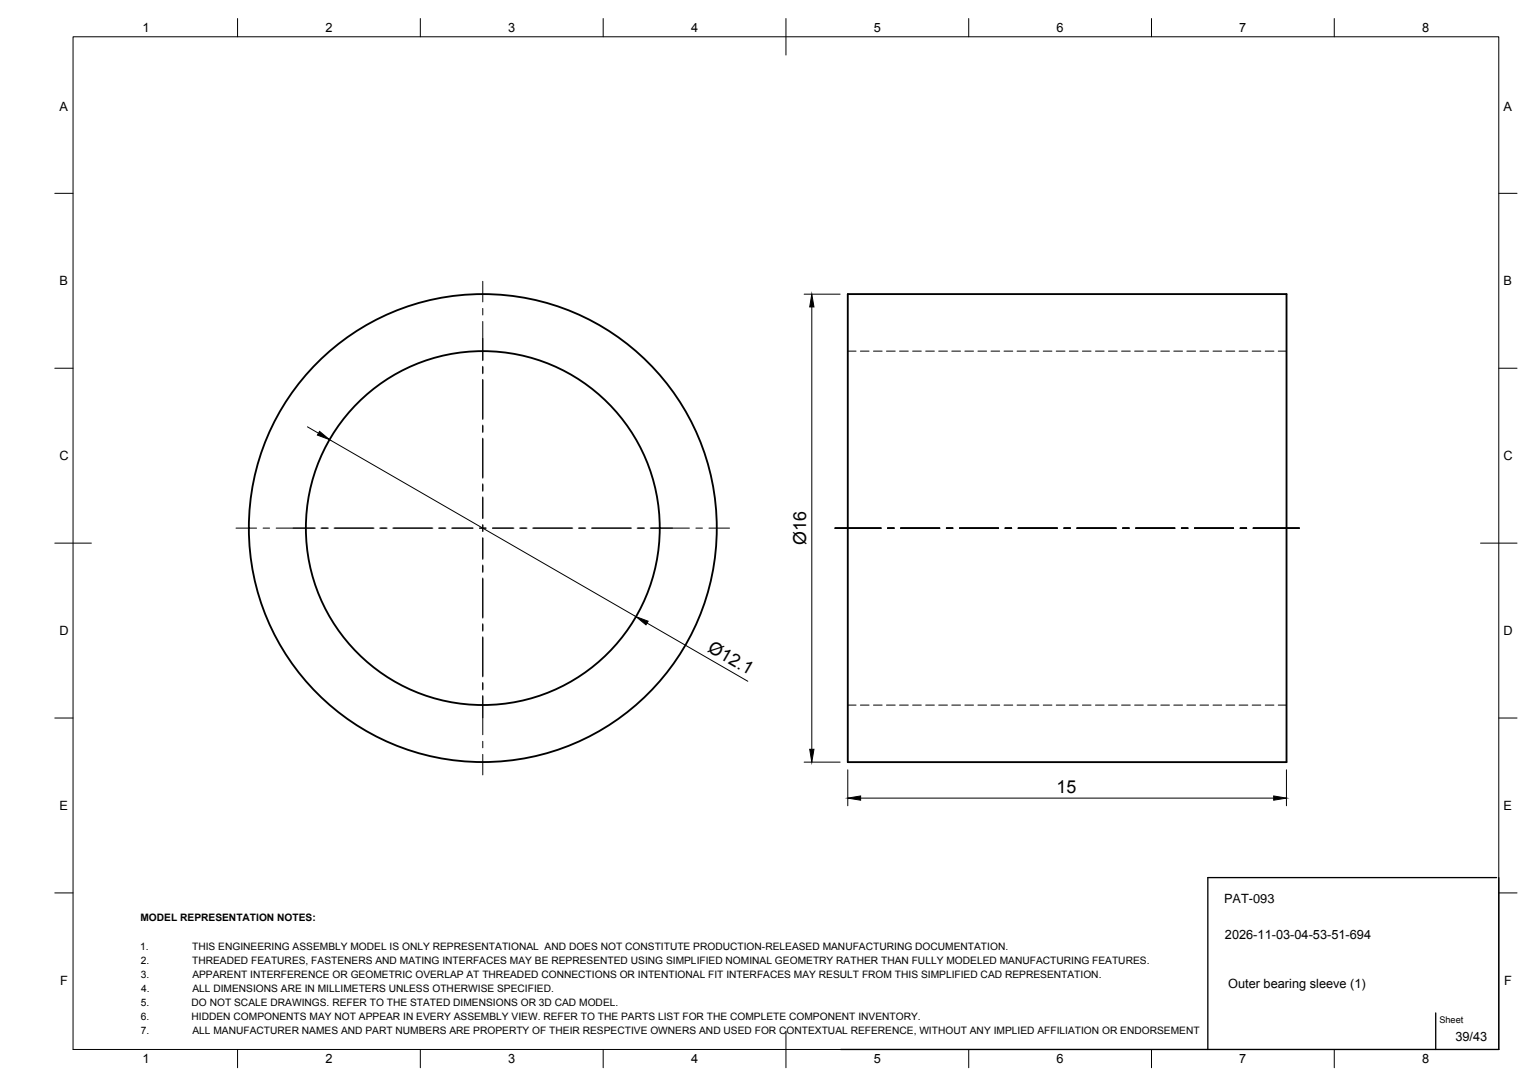
ISO-10303-21;
HEADER;
/* Generated by software containing ST-Developer
 * from STEP Tools, Inc. (www.steptools.com) 
 */

FILE_DESCRIPTION(
/* description */ ('Self-centering screw clamp'),
/* implementation_level */ '2;1');

FILE_NAME(
/* name */ 'Outer bearing sleeve (1).step',
/* time_stamp */ '2026-10-28T03:25:31-07:00',
/* author */ (''),
/* organization */ (''),
/* preprocessor_version */ 'ST-DEVELOPER v20.2',
/* originating_system */ 'Autodesk Translation Framework v15.17.0.0',
/* authorisation */ '');

FILE_SCHEMA (('AUTOMOTIVE_DESIGN { 1 0 10303 214 3 1 1 }'));
ENDSEC;

DATA;
#10=MECHANICAL_DESIGN_GEOMETRIC_PRESENTATION_REPRESENTATION('',(#665),#16799);
#576=SHAPE_REPRESENTATION_RELATIONSHIP('SRR','None',#17054,#617);
#617=ADVANCED_BREP_SHAPE_REPRESENTATION('',(#712),#16792);
#665=STYLED_ITEM('',(#17326),#712);
#712=MANIFOLD_SOLID_BREP('Body1',#9117);
#1001=FACE_BOUND('',#2510,.T.);
#1002=FACE_BOUND('',#2512,.T.);
#1238=PLANE('',#10551);
#1239=PLANE('',#10552);
#1720=FACE_OUTER_BOUND('',#2507,.T.);
#1721=FACE_OUTER_BOUND('',#2508,.T.);
#1722=FACE_OUTER_BOUND('',#2509,.T.);
#1723=FACE_OUTER_BOUND('',#2511,.T.);
#2507=EDGE_LOOP('',(#8121,#8122,#8123,#8124));
#2508=EDGE_LOOP('',(#8125,#8126,#8127,#8128));
#2509=EDGE_LOOP('',(#8129));
#2510=EDGE_LOOP('',(#8130));
#2511=EDGE_LOOP('',(#8131));
#2512=EDGE_LOOP('',(#8132));
#3084=LINE('',#16225,#3657);
#3085=LINE('',#16231,#3658);
#3657=VECTOR('',#13199,0.605);
#3658=VECTOR('',#13206,0.8);
#4195=CIRCLE('',#10546,0.605);
#4196=CIRCLE('',#10547,0.605);
#4197=CIRCLE('',#10549,0.8);
#4198=CIRCLE('',#10550,0.8);
#4900=VERTEX_POINT('',#16222);
#4901=VERTEX_POINT('',#16224);
#4902=VERTEX_POINT('',#16228);
#4903=VERTEX_POINT('',#16230);
#5985=EDGE_CURVE('',#4900,#4900,#4195,.T.);
#5986=EDGE_CURVE('',#4900,#4901,#3084,.T.);
#5987=EDGE_CURVE('',#4901,#4901,#4196,.T.);
#5988=EDGE_CURVE('',#4902,#4902,#4197,.T.);
#5989=EDGE_CURVE('',#4902,#4903,#3085,.T.);
#5990=EDGE_CURVE('',#4903,#4903,#4198,.T.);
#8121=ORIENTED_EDGE('',*,*,#5985,.F.);
#8122=ORIENTED_EDGE('',*,*,#5986,.T.);
#8123=ORIENTED_EDGE('',*,*,#5987,.T.);
#8124=ORIENTED_EDGE('',*,*,#5986,.F.);
#8125=ORIENTED_EDGE('',*,*,#5988,.F.);
#8126=ORIENTED_EDGE('',*,*,#5989,.T.);
#8127=ORIENTED_EDGE('',*,*,#5990,.T.);
#8128=ORIENTED_EDGE('',*,*,#5989,.F.);
#8129=ORIENTED_EDGE('',*,*,#5988,.T.);
#8130=ORIENTED_EDGE('',*,*,#5985,.T.);
#8131=ORIENTED_EDGE('',*,*,#5990,.F.);
#8132=ORIENTED_EDGE('',*,*,#5987,.F.);
#8555=CYLINDRICAL_SURFACE('',#10545,0.605);
#8556=CYLINDRICAL_SURFACE('',#10548,0.8);
#9018=ADVANCED_FACE('',(#1720),#8555,.F.);
#9019=ADVANCED_FACE('',(#1721),#8556,.T.);
#9020=ADVANCED_FACE('',(#1722,#1001),#1238,.T.);
#9021=ADVANCED_FACE('',(#1723,#1002),#1239,.F.);
#9117=CLOSED_SHELL('',(#9018,#9019,#9020,#9021));
#10544=AXIS2_PLACEMENT_3D('',#16220,#13193,#13194);
#10545=AXIS2_PLACEMENT_3D('',#16221,#13195,#13196);
#10546=AXIS2_PLACEMENT_3D('',#16223,#13197,#13198);
#10547=AXIS2_PLACEMENT_3D('',#16226,#13200,#13201);
#10548=AXIS2_PLACEMENT_3D('',#16227,#13202,#13203);
#10549=AXIS2_PLACEMENT_3D('',#16229,#13204,#13205);
#10550=AXIS2_PLACEMENT_3D('',#16232,#13207,#13208);
#10551=AXIS2_PLACEMENT_3D('',#16233,#13209,#13210);
#10552=AXIS2_PLACEMENT_3D('',#16234,#13211,#13212);
#13193=DIRECTION('axis',(0.,0.,1.));
#13194=DIRECTION('refdir',(1.,0.,0.));
#13195=DIRECTION('center_axis',(1.,0.,0.));
#13196=DIRECTION('ref_axis',(0.,0.,-1.));
#13197=DIRECTION('center_axis',(-1.,0.,0.));
#13198=DIRECTION('ref_axis',(0.,0.,-1.));
#13199=DIRECTION('',(-1.,0.,0.));
#13200=DIRECTION('center_axis',(-1.,0.,0.));
#13201=DIRECTION('ref_axis',(0.,0.,-1.));
#13202=DIRECTION('center_axis',(1.,0.,0.));
#13203=DIRECTION('ref_axis',(0.,0.,-1.));
#13204=DIRECTION('center_axis',(1.,0.,0.));
#13205=DIRECTION('ref_axis',(0.,0.,-1.));
#13206=DIRECTION('',(-1.,0.,0.));
#13207=DIRECTION('center_axis',(1.,0.,0.));
#13208=DIRECTION('ref_axis',(0.,0.,-1.));
#13209=DIRECTION('center_axis',(1.,0.,0.));
#13210=DIRECTION('ref_axis',(0.,0.,-1.));
#13211=DIRECTION('center_axis',(1.,0.,0.));
#13212=DIRECTION('ref_axis',(0.,0.,-1.));
#16220=CARTESIAN_POINT('',(0.,0.,0.));
#16221=CARTESIAN_POINT('Origin',(12.,0.,4.));
#16222=CARTESIAN_POINT('',(13.5,-7.40911313484149E-17,4.605));
#16223=CARTESIAN_POINT('Origin',(13.5,0.,4.));
#16224=CARTESIAN_POINT('',(12.,-7.40911313484149E-17,4.605));
#16225=CARTESIAN_POINT('',(12.,-7.40911313484149E-17,4.605));
#16226=CARTESIAN_POINT('Origin',(12.,0.,4.));
#16227=CARTESIAN_POINT('Origin',(12.,0.,4.));
#16228=CARTESIAN_POINT('',(13.5,-9.79717439317882E-17,4.8));
#16229=CARTESIAN_POINT('Origin',(13.5,0.,4.));
#16230=CARTESIAN_POINT('',(12.,-9.79717439317882E-17,4.8));
#16231=CARTESIAN_POINT('',(12.,-9.79717439317882E-17,4.8));
#16232=CARTESIAN_POINT('Origin',(12.,0.,4.));
#16233=CARTESIAN_POINT('Origin',(13.5,0.,4.));
#16234=CARTESIAN_POINT('Origin',(12.,0.,4.));
#16743=UNCERTAINTY_MEASURE_WITH_UNIT(LENGTH_MEASURE(0.001),#16800,
'DISTANCE_ACCURACY_VALUE',
'Maximum model space distance between geometric entities at asserted c
onnectivities');
#16750=UNCERTAINTY_MEASURE_WITH_UNIT(LENGTH_MEASURE(0.001),#16800,
'DISTANCE_ACCURACY_VALUE',
'Maximum model space distance between geometric entities at asserted c
onnectivities');
#16792=(
GEOMETRIC_REPRESENTATION_CONTEXT(3)
GLOBAL_UNCERTAINTY_ASSIGNED_CONTEXT((#16743))
GLOBAL_UNIT_ASSIGNED_CONTEXT((#16800,#16802,#16803))
REPRESENTATION_CONTEXT('','3D')
);
#16799=(
GEOMETRIC_REPRESENTATION_CONTEXT(3)
GLOBAL_UNCERTAINTY_ASSIGNED_CONTEXT((#16750))
GLOBAL_UNIT_ASSIGNED_CONTEXT((#16800,#16802,#16803))
REPRESENTATION_CONTEXT('','3D')
);
#16800=(
LENGTH_UNIT()
NAMED_UNIT(*)
SI_UNIT(.CENTI.,.METRE.)
);
#16802=(
NAMED_UNIT(*)
PLANE_ANGLE_UNIT()
SI_UNIT($,.RADIAN.)
);
#16803=(
NAMED_UNIT(*)
SI_UNIT($,.STERADIAN.)
SOLID_ANGLE_UNIT()
);
#16845=SHAPE_DEFINITION_REPRESENTATION(#16900,#17054);
#16900=PRODUCT_DEFINITION_SHAPE('',$,#17103);
#17054=SHAPE_REPRESENTATION('',(#10544),#16792);
#17061=PRODUCT_DEFINITION_CONTEXT('part definition',#17207,'design');
#17103=PRODUCT_DEFINITION('Outer bearing sleeve (1)',
'Outer bearing sleeve (1)',#17151,#17061);
#17151=PRODUCT_DEFINITION_FORMATION('',$,#17250);
#17207=APPLICATION_CONTEXT(
'Core Data for Automotive Mechanical Design Process');
#17208=PRODUCT_CONTEXT('part definition',#17207,'mechanical');
#17250=PRODUCT('Outer bearing sleeve (1)','Outer bearing sleeve (1)',
'Outer bearing sleeve (1)',(#17208));
#17320=COLOUR_RGB('Grey',0.48,0.52,0.57);
#17321=FILL_AREA_STYLE_COLOUR('',#17320);
#17322=FILL_AREA_STYLE('',(#17321));
#17323=SURFACE_STYLE_FILL_AREA(#17322);
#17324=SURFACE_SIDE_STYLE('',(#17323));
#17325=SURFACE_STYLE_USAGE(.BOTH.,#17324);
#17326=PRESENTATION_STYLE_ASSIGNMENT((#17325));
ENDSEC;
END-ISO-10303-21;
